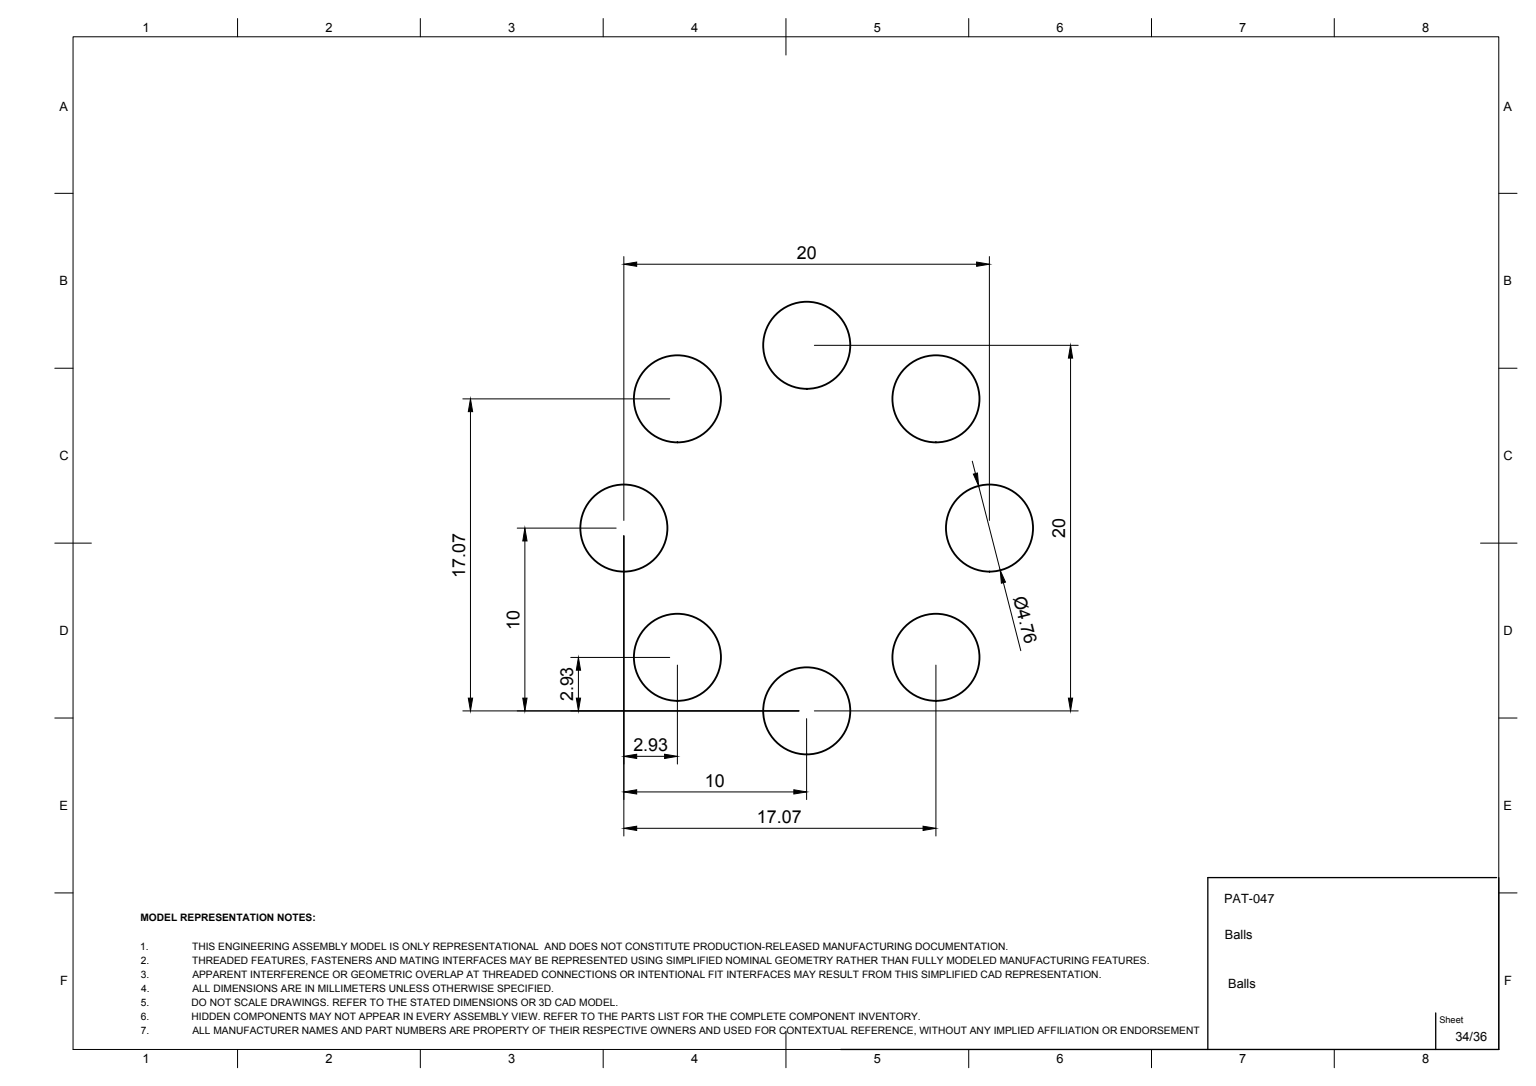
ISO-10303-21;
HEADER;
/* Generated by software containing ST-Developer
 * from STEP Tools, Inc. (www.steptools.com) 
 */

FILE_DESCRIPTION(
/* description */ ('Gravity roller conveyor section'),
/* implementation_level */ '2;1');

FILE_NAME(
/* name */ 'Balls.step',
/* time_stamp */ '2026-11-02T07:43:02-08:00',
/* author */ (''),
/* organization */ (''),
/* preprocessor_version */ 'ST-DEVELOPER v20.2',
/* originating_system */ 'Autodesk Translation Framework v15.17.0.0',
/* authorisation */ '');

FILE_SCHEMA (('AUTOMOTIVE_DESIGN { 1 0 10303 214 3 1 1 }'));
ENDSEC;

DATA;
#10=MECHANICAL_DESIGN_GEOMETRIC_PRESENTATION_REPRESENTATION('',(#554,#555,#556,#557,#558,#559,#560,#561),#13821);
#389=SPHERICAL_SURFACE('',#8525,0.23815);
#390=SPHERICAL_SURFACE('',#8527,0.23815);
#391=SPHERICAL_SURFACE('',#8529,0.23815);
#392=SPHERICAL_SURFACE('',#8531,0.23815);
#393=SPHERICAL_SURFACE('',#8533,0.23815);
#394=SPHERICAL_SURFACE('',#8535,0.23815);
#395=SPHERICAL_SURFACE('',#8537,0.23815);
#396=SPHERICAL_SURFACE('',#8539,0.23815);
#486=SHAPE_REPRESENTATION_RELATIONSHIP('SRR','None',#14025,#520);
#520=ADVANCED_BREP_SHAPE_REPRESENTATION('',(#594,#595,#596,#597,#598,#599,
#600,#601),#13812);
#554=STYLED_ITEM('',(#14191),#594);
#555=STYLED_ITEM('',(#14191),#595);
#556=STYLED_ITEM('',(#14191),#596);
#557=STYLED_ITEM('',(#14191),#597);
#558=STYLED_ITEM('',(#14191),#598);
#559=STYLED_ITEM('',(#14191),#599);
#560=STYLED_ITEM('',(#14191),#600);
#561=STYLED_ITEM('',(#14191),#601);
#594=MANIFOLD_SOLID_BREP('Body1',#7654);
#595=MANIFOLD_SOLID_BREP('Body2',#7655);
#596=MANIFOLD_SOLID_BREP('Body3',#7656);
#597=MANIFOLD_SOLID_BREP('Body4',#7657);
#598=MANIFOLD_SOLID_BREP('Body5',#7658);
#599=MANIFOLD_SOLID_BREP('Body6',#7659);
#600=MANIFOLD_SOLID_BREP('Body7',#7660);
#601=MANIFOLD_SOLID_BREP('Body8',#7661);
#1324=FACE_OUTER_BOUND('',#1816,.T.);
#1325=FACE_OUTER_BOUND('',#1817,.T.);
#1326=FACE_OUTER_BOUND('',#1818,.T.);
#1327=FACE_OUTER_BOUND('',#1819,.T.);
#1328=FACE_OUTER_BOUND('',#1820,.T.);
#1329=FACE_OUTER_BOUND('',#1821,.T.);
#1330=FACE_OUTER_BOUND('',#1822,.T.);
#1331=FACE_OUTER_BOUND('',#1823,.T.);
#1816=EDGE_LOOP('',(#6706,#6707));
#1817=EDGE_LOOP('',(#6708,#6709));
#1818=EDGE_LOOP('',(#6710,#6711));
#1819=EDGE_LOOP('',(#6712,#6713));
#1820=EDGE_LOOP('',(#6714,#6715));
#1821=EDGE_LOOP('',(#6716,#6717));
#1822=EDGE_LOOP('',(#6718,#6719));
#1823=EDGE_LOOP('',(#6720,#6721));
#3504=CIRCLE('',#8526,0.23815);
#3505=CIRCLE('',#8528,0.23815);
#3506=CIRCLE('',#8530,0.23815);
#3507=CIRCLE('',#8532,0.23815);
#3508=CIRCLE('',#8534,0.23815);
#3509=CIRCLE('',#8536,0.23815);
#3510=CIRCLE('',#8538,0.23815);
#3511=CIRCLE('',#8540,0.23815);
#4088=VERTEX_POINT('',#12841);
#4089=VERTEX_POINT('',#12842);
#4090=VERTEX_POINT('',#12845);
#4091=VERTEX_POINT('',#12846);
#4092=VERTEX_POINT('',#12849);
#4093=VERTEX_POINT('',#12850);
#4094=VERTEX_POINT('',#12853);
#4095=VERTEX_POINT('',#12854);
#4096=VERTEX_POINT('',#12857);
#4097=VERTEX_POINT('',#12858);
#4098=VERTEX_POINT('',#12861);
#4099=VERTEX_POINT('',#12862);
#4100=VERTEX_POINT('',#12865);
#4101=VERTEX_POINT('',#12866);
#4102=VERTEX_POINT('',#12869);
#4103=VERTEX_POINT('',#12870);
#4990=EDGE_CURVE('',#4088,#4089,#3504,.T.);
#4991=EDGE_CURVE('',#4090,#4091,#3505,.T.);
#4992=EDGE_CURVE('',#4092,#4093,#3506,.T.);
#4993=EDGE_CURVE('',#4094,#4095,#3507,.T.);
#4994=EDGE_CURVE('',#4096,#4097,#3508,.T.);
#4995=EDGE_CURVE('',#4098,#4099,#3509,.T.);
#4996=EDGE_CURVE('',#4100,#4101,#3510,.T.);
#4997=EDGE_CURVE('',#4102,#4103,#3511,.T.);
#6706=ORIENTED_EDGE('',*,*,#4990,.T.);
#6707=ORIENTED_EDGE('',*,*,#4990,.F.);
#6708=ORIENTED_EDGE('',*,*,#4991,.T.);
#6709=ORIENTED_EDGE('',*,*,#4991,.F.);
#6710=ORIENTED_EDGE('',*,*,#4992,.T.);
#6711=ORIENTED_EDGE('',*,*,#4992,.F.);
#6712=ORIENTED_EDGE('',*,*,#4993,.T.);
#6713=ORIENTED_EDGE('',*,*,#4993,.F.);
#6714=ORIENTED_EDGE('',*,*,#4994,.T.);
#6715=ORIENTED_EDGE('',*,*,#4994,.F.);
#6716=ORIENTED_EDGE('',*,*,#4995,.T.);
#6717=ORIENTED_EDGE('',*,*,#4995,.F.);
#6718=ORIENTED_EDGE('',*,*,#4996,.T.);
#6719=ORIENTED_EDGE('',*,*,#4996,.F.);
#6720=ORIENTED_EDGE('',*,*,#4997,.T.);
#6721=ORIENTED_EDGE('',*,*,#4997,.F.);
#7525=ADVANCED_FACE('',(#1324),#389,.T.);
#7526=ADVANCED_FACE('',(#1325),#390,.T.);
#7527=ADVANCED_FACE('',(#1326),#391,.T.);
#7528=ADVANCED_FACE('',(#1327),#392,.T.);
#7529=ADVANCED_FACE('',(#1328),#393,.T.);
#7530=ADVANCED_FACE('',(#1329),#394,.T.);
#7531=ADVANCED_FACE('',(#1330),#395,.T.);
#7532=ADVANCED_FACE('',(#1331),#396,.T.);
#7654=CLOSED_SHELL('',(#7525));
#7655=CLOSED_SHELL('',(#7526));
#7656=CLOSED_SHELL('',(#7527));
#7657=CLOSED_SHELL('',(#7528));
#7658=CLOSED_SHELL('',(#7529));
#7659=CLOSED_SHELL('',(#7530));
#7660=CLOSED_SHELL('',(#7531));
#7661=CLOSED_SHELL('',(#7532));
#8524=AXIS2_PLACEMENT_3D('',#12839,#10381,#10382);
#8525=AXIS2_PLACEMENT_3D('',#12840,#10383,#10384);
#8526=AXIS2_PLACEMENT_3D('',#12843,#10385,#10386);
#8527=AXIS2_PLACEMENT_3D('',#12844,#10387,#10388);
#8528=AXIS2_PLACEMENT_3D('',#12847,#10389,#10390);
#8529=AXIS2_PLACEMENT_3D('',#12848,#10391,#10392);
#8530=AXIS2_PLACEMENT_3D('',#12851,#10393,#10394);
#8531=AXIS2_PLACEMENT_3D('',#12852,#10395,#10396);
#8532=AXIS2_PLACEMENT_3D('',#12855,#10397,#10398);
#8533=AXIS2_PLACEMENT_3D('',#12856,#10399,#10400);
#8534=AXIS2_PLACEMENT_3D('',#12859,#10401,#10402);
#8535=AXIS2_PLACEMENT_3D('',#12860,#10403,#10404);
#8536=AXIS2_PLACEMENT_3D('',#12863,#10405,#10406);
#8537=AXIS2_PLACEMENT_3D('',#12864,#10407,#10408);
#8538=AXIS2_PLACEMENT_3D('',#12867,#10409,#10410);
#8539=AXIS2_PLACEMENT_3D('',#12868,#10411,#10412);
#8540=AXIS2_PLACEMENT_3D('',#12871,#10413,#10414);
#10381=DIRECTION('axis',(0.,0.,1.));
#10382=DIRECTION('refdir',(1.,0.,0.));
#10383=DIRECTION('center_axis',(0.,0.,1.));
#10384=DIRECTION('ref_axis',(1.,0.,0.));
#10385=DIRECTION('center_axis',(1.22464679914735E-16,-1.,0.));
#10386=DIRECTION('ref_axis',(-1.,-1.22464679914735E-16,0.));
#10387=DIRECTION('center_axis',(0.707106781186548,0.,0.707106781186548));
#10388=DIRECTION('ref_axis',(0.707106781186548,0.,-0.707106781186548));
#10389=DIRECTION('center_axis',(8.65956056235494E-17,-1.,-8.65956056235493E-17));
#10390=DIRECTION('ref_axis',(-0.707106781186547,-1.22464679914735E-16,0.707106781186547));
#10391=DIRECTION('center_axis',(1.,0.,0.));
#10392=DIRECTION('ref_axis',(6.12323399573676E-17,0.,-1.));
#10393=DIRECTION('center_axis',(7.49879891330929E-33,-1.,-1.22464679914735E-16));
#10394=DIRECTION('ref_axis',(-6.12323399573676E-17,-1.22464679914735E-16,
1.));
#10395=DIRECTION('center_axis',(0.707106781186548,0.,-0.707106781186548));
#10396=DIRECTION('ref_axis',(-0.707106781186548,0.,-0.707106781186548));
#10397=DIRECTION('center_axis',(-8.65956056235493E-17,-1.,-8.65956056235494E-17));
#10398=DIRECTION('ref_axis',(0.707106781186547,-1.22464679914735E-16,0.707106781186547));
#10399=DIRECTION('center_axis',(0.,0.,-1.));
#10400=DIRECTION('ref_axis',(-1.,0.,-1.22464679914735E-16));
#10401=DIRECTION('center_axis',(-1.22464679914735E-16,-1.,-1.49975978266186E-32));
#10402=DIRECTION('ref_axis',(1.,-1.22464679914735E-16,1.22464679914735E-16));
#10403=DIRECTION('center_axis',(-0.707106781186547,0.,-0.707106781186548));
#10404=DIRECTION('ref_axis',(-0.707106781186548,0.,0.707106781186547));
#10405=DIRECTION('center_axis',(-8.65956056235493E-17,-1.,8.65956056235493E-17));
#10406=DIRECTION('ref_axis',(0.707106781186548,-1.22464679914735E-16,-0.707106781186547));
#10407=DIRECTION('center_axis',(-1.,0.,0.));
#10408=DIRECTION('ref_axis',(-1.83697019872103E-16,0.,1.));
#10409=DIRECTION('center_axis',(-2.24963967399279E-32,-1.,1.22464679914735E-16));
#10410=DIRECTION('ref_axis',(1.83697019872103E-16,-1.22464679914735E-16,
-1.));
#10411=DIRECTION('center_axis',(-0.707106781186548,0.,0.707106781186548));
#10412=DIRECTION('ref_axis',(0.707106781186547,0.,0.707106781186548));
#10413=DIRECTION('center_axis',(8.65956056235493E-17,-1.,8.65956056235493E-17));
#10414=DIRECTION('ref_axis',(-0.707106781186547,-1.22464679914735E-16,-0.707106781186548));
#12839=CARTESIAN_POINT('',(0.,0.,0.));
#12840=CARTESIAN_POINT('Origin',(1.,0.,0.));
#12841=CARTESIAN_POINT('',(1.,-1.78583896120461E-33,0.23815));
#12842=CARTESIAN_POINT('',(1.,-1.78583896120461E-33,-0.23815));
#12843=CARTESIAN_POINT('Origin',(1.,0.,0.));
#12844=CARTESIAN_POINT('Origin',(0.707106781186548,0.,-0.707106781186547));
#12845=CARTESIAN_POINT('',(0.875504261126124,-1.78583896120461E-33,-0.538709301246971));
#12846=CARTESIAN_POINT('',(0.538709301246971,-1.78583896120461E-33,-0.875504261126124));
#12847=CARTESIAN_POINT('Origin',(0.707106781186548,0.,-0.707106781186547));
#12848=CARTESIAN_POINT('Origin',(6.12323399573677E-17,0.,-1.));
#12849=CARTESIAN_POINT('',(0.23815,-1.78583896120461E-33,-1.));
#12850=CARTESIAN_POINT('',(-0.23815,-1.78583896120461E-33,-1.));
#12851=CARTESIAN_POINT('Origin',(6.12323399573677E-17,0.,-1.));
#12852=CARTESIAN_POINT('Origin',(-0.707106781186547,0.,-0.707106781186548));
#12853=CARTESIAN_POINT('',(-0.538709301246971,-1.78583896120461E-33,-0.875504261126124));
#12854=CARTESIAN_POINT('',(-0.875504261126124,-1.78583896120461E-33,-0.538709301246971));
#12855=CARTESIAN_POINT('Origin',(-0.707106781186547,0.,-0.707106781186548));
#12856=CARTESIAN_POINT('Origin',(-1.,0.,-1.22464679914735E-16));
#12857=CARTESIAN_POINT('',(-1.,-1.78583896120461E-33,-0.23815));
#12858=CARTESIAN_POINT('',(-1.,-1.78583896120461E-33,0.23815));
#12859=CARTESIAN_POINT('Origin',(-1.,0.,-1.22464679914735E-16));
#12860=CARTESIAN_POINT('Origin',(-0.707106781186548,0.,0.707106781186547));
#12861=CARTESIAN_POINT('',(-0.875504261126124,-7.94881478324376E-33,0.538709301246971));
#12862=CARTESIAN_POINT('',(-0.538709301246971,4.37713686083455E-33,0.875504261126124));
#12863=CARTESIAN_POINT('Origin',(-0.707106781186548,0.,0.707106781186547));
#12864=CARTESIAN_POINT('Origin',(-1.83697019872103E-16,0.,1.));
#12865=CARTESIAN_POINT('',(-0.23815,-1.78583896120461E-33,1.));
#12866=CARTESIAN_POINT('',(0.23815,-1.78583896120461E-33,1.));
#12867=CARTESIAN_POINT('Origin',(-1.83697019872103E-16,0.,1.));
#12868=CARTESIAN_POINT('Origin',(0.707106781186547,0.,0.707106781186548));
#12869=CARTESIAN_POINT('',(0.538709301246971,-4.86732687222419E-33,0.875504261126124));
#12870=CARTESIAN_POINT('',(0.875504261126124,1.29564894981497E-33,0.538709301246971));
#12871=CARTESIAN_POINT('Origin',(0.707106781186547,0.,0.707106781186548));
#13773=UNCERTAINTY_MEASURE_WITH_UNIT(LENGTH_MEASURE(0.001),#13822,
'DISTANCE_ACCURACY_VALUE',
'Maximum model space distance between geometric entities at asserted c
onnectivities');
#13782=UNCERTAINTY_MEASURE_WITH_UNIT(LENGTH_MEASURE(0.001),#13822,
'DISTANCE_ACCURACY_VALUE',
'Maximum model space distance between geometric entities at asserted c
onnectivities');
#13812=(
GEOMETRIC_REPRESENTATION_CONTEXT(3)
GLOBAL_UNCERTAINTY_ASSIGNED_CONTEXT((#13773))
GLOBAL_UNIT_ASSIGNED_CONTEXT((#13822,#13824,#13825))
REPRESENTATION_CONTEXT('','3D')
);
#13821=(
GEOMETRIC_REPRESENTATION_CONTEXT(3)
GLOBAL_UNCERTAINTY_ASSIGNED_CONTEXT((#13782))
GLOBAL_UNIT_ASSIGNED_CONTEXT((#13822,#13824,#13825))
REPRESENTATION_CONTEXT('','3D')
);
#13822=(
LENGTH_UNIT()
NAMED_UNIT(*)
SI_UNIT(.CENTI.,.METRE.)
);
#13824=(
NAMED_UNIT(*)
PLANE_ANGLE_UNIT()
SI_UNIT($,.RADIAN.)
);
#13825=(
NAMED_UNIT(*)
SI_UNIT($,.STERADIAN.)
SOLID_ANGLE_UNIT()
);
#13855=SHAPE_DEFINITION_REPRESENTATION(#13893,#14025);
#13893=PRODUCT_DEFINITION_SHAPE('',$,#14064);
#14025=SHAPE_REPRESENTATION('',(#8524),#13812);
#14034=PRODUCT_DEFINITION_CONTEXT('part definition',#14150,'design');
#14064=PRODUCT_DEFINITION('Balls','Balls',#14102,#14034);
#14102=PRODUCT_DEFINITION_FORMATION('',$,#14181);
#14150=APPLICATION_CONTEXT(
'Core Data for Automotive Mechanical Design Process');
#14151=PRODUCT_CONTEXT('part definition',#14150,'mechanical');
#14181=PRODUCT('Balls','Balls','Balls',(#14151));
#14191=PRESENTATION_STYLE_ASSIGNMENT((#14196));
#14196=SURFACE_STYLE_USAGE(.BOTH.,#14201);
#14201=SURFACE_SIDE_STYLE('',(#14206));
#14206=SURFACE_STYLE_FILL_AREA(#14211);
#14211=FILL_AREA_STYLE('CAD Library Painted - Steel gray',(#14216));
#14216=FILL_AREA_STYLE_COLOUR('CAD Library Painted - Steel gray',#14221);
#14221=COLOUR_RGB('CAD Library Painted - Steel gray',0.592156862745098,
0.631372549019608,0.67843137254902);
ENDSEC;
END-ISO-10303-21;
